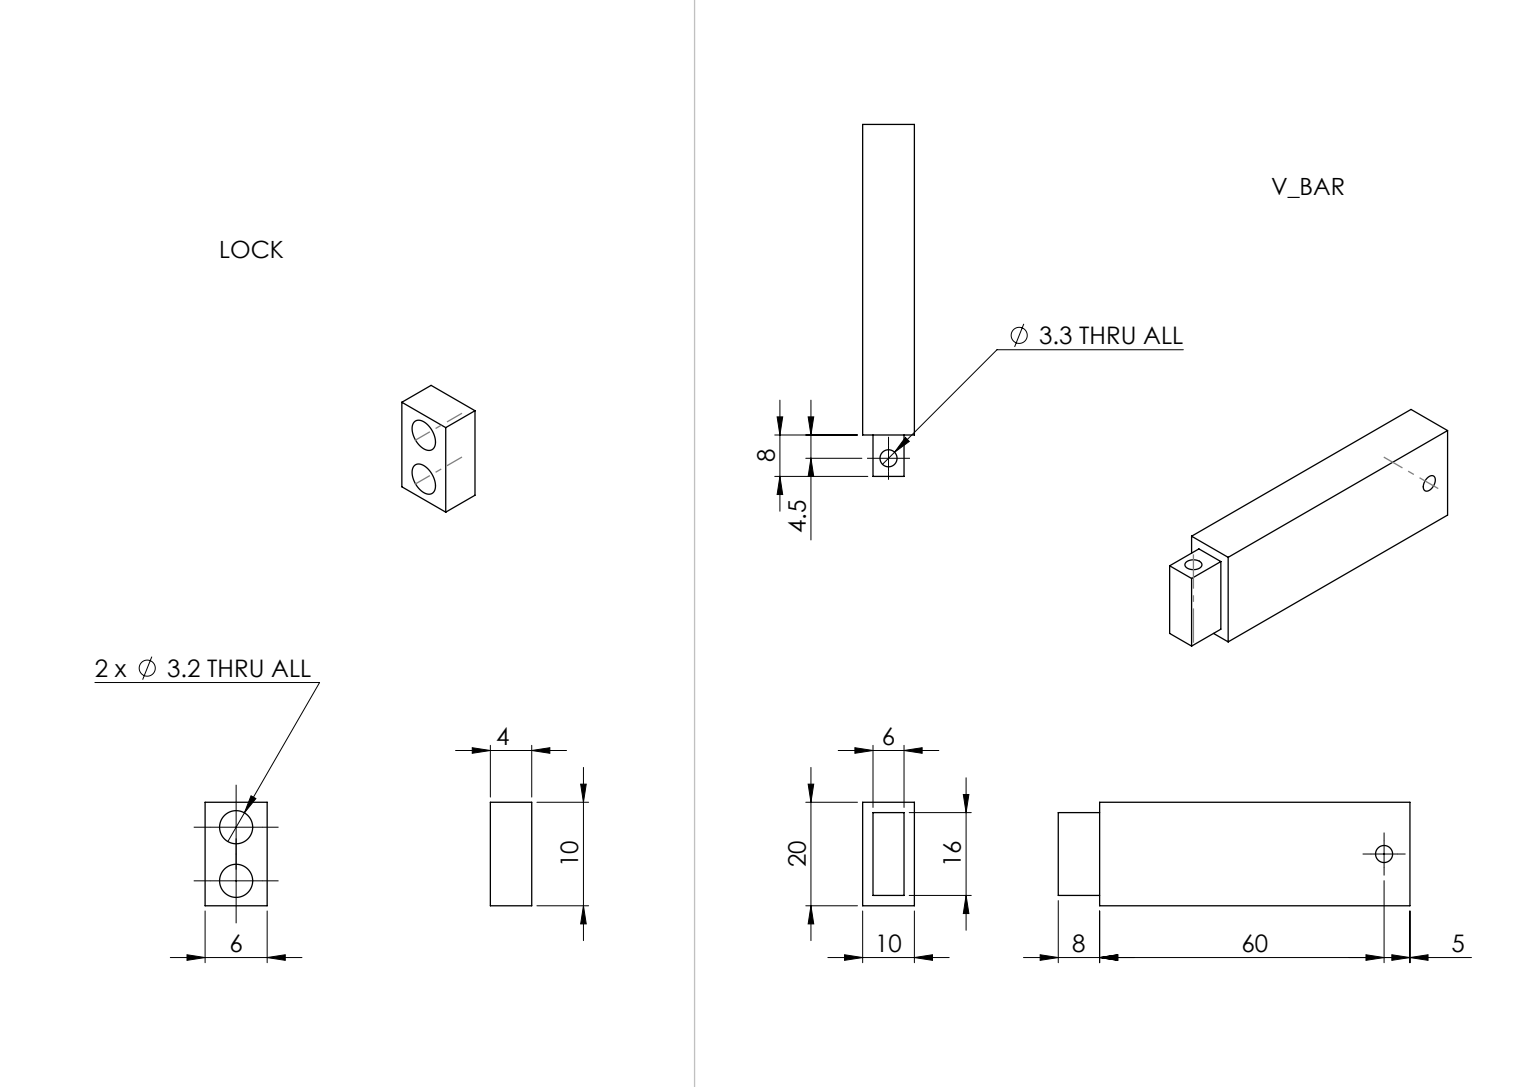
ISO-10303-21;
HEADER;
FILE_DESCRIPTION (('STEP AP214'),
    '1' );
FILE_NAME ('lock.step',
    '2026-10-08T12:12:07',
    ( '' ),
    ( '' ),
    'SwSTEP 2.0',
    'SolidWorks 2026',
    '' );
FILE_SCHEMA (( 'AUTOMOTIVE_DESIGN' ));
ENDSEC;

DATA;
#16=EDGE_LOOP ( 'NONE', ( #282, #7065, #6159, #322 ) ) ;
#17=ADVANCED_FACE ( 'NONE', ( #5328 ), #856, .F. ) ;
#69=CYLINDRICAL_SURFACE ( 'NONE', #6742, 1.599999999999992983 ) ;
#73=EDGE_LOOP ( 'NONE', ( #3445, #4824, #2962, #715 ) ) ;
#74=FACE_OUTER_BOUND ( 'NONE', #4146, .T. ) ;
#91=SURFACE_SIDE_STYLE ('',( #6493 ) ) ;
#113=DIRECTION ( 'NONE',  ( -1.734723475976806848E-16, 1.000000000000000000, -0.000000000000000000 ) ) ;
#141=SURFACE_STYLE_USAGE ( .BOTH. , #5841 ) ;
#160=ORIENTED_EDGE ( 'NONE', *, *, #1858, .F. ) ;
#167=EDGE_CURVE ( 'NONE', #3524, #3495, #1661, .T. ) ;
#171=FACE_BOUND ( 'NONE', #7717, .T. ) ;
#177=CARTESIAN_POINT ( 'NONE',  ( 1.599999999999986988, 42.68016229225776925, 0.000000000000000000 ) ) ;
#236=CARTESIAN_POINT ( 'NONE',  ( -3.000000000000000888, 45.09008114612887397, 4.000000000000000000 ) ) ;
#237=PRODUCT_CONTEXT ( 'NONE', #7877, 'mechanical' ) ;
#282=ORIENTED_EDGE ( 'NONE', *, *, #5845, .T. ) ;
#290=FILL_AREA_STYLE_COLOUR ( '', #5069 ) ;
#322=ORIENTED_EDGE ( 'NONE', *, *, #4660, .T. ) ;
#339=ORIENTED_EDGE ( 'NONE', *, *, #6913, .F. ) ;
#436=( GEOMETRIC_REPRESENTATION_CONTEXT ( 3 ) GLOBAL_UNCERTAINTY_ASSIGNED_CONTEXT ( ( #3628 ) ) GLOBAL_UNIT_ASSIGNED_CONTEXT ( ( #6999, #3191, #7744 ) ) REPRESENTATION_CONTEXT ( 'NONE', 'WORKASPACE' ) );
#515=CARTESIAN_POINT ( 'NONE',  ( -3.000000000000000888, 45.09008114612887397, 4.000000000000000000 ) ) ;
#540=( GEOMETRIC_REPRESENTATION_CONTEXT ( 3 ) GLOBAL_UNCERTAINTY_ASSIGNED_CONTEXT ( ( #3548 ) ) GLOBAL_UNIT_ASSIGNED_CONTEXT ( ( #3306, #2837, #2061 ) ) REPRESENTATION_CONTEXT ( 'NONE', 'WORKASPACE' ) );
#548=LINE ( 'NONE', #1806, #3702 ) ;
#561=DIRECTION ( 'NONE',  ( -0.000000000000000000, -0.000000000000000000, 1.000000000000000000 ) ) ;
#575=LINE ( 'NONE', #3747, #3853 ) ;
#588=EDGE_LOOP ( 'NONE', ( #3671, #2915, #1768, #4961 ) ) ;
#600=PRODUCT ( 'lock', 'lock', '', ( #237 ) ) ;
#604=VERTEX_POINT ( 'NONE', #1255 ) ;
#616=CARTESIAN_POINT ( 'NONE',  ( -1.600000000000010969, 42.68016229225776925, 0.000000000000000000 ) ) ;
#634=ADVANCED_FACE ( 'NONE', ( #74 ), #4574, .F. ) ;
#637=DIRECTION ( 'NONE',  ( -0.000000000000000000, -0.000000000000000000, 1.000000000000000000 ) ) ;
#640=VECTOR ( 'NONE', #5019, 1000.000000000000000 ) ;
#673=ORIENTED_EDGE ( 'NONE', *, *, #2621, .F. ) ;
#715=ORIENTED_EDGE ( 'NONE', *, *, #2234, .T. ) ;
#791=AXIS2_PLACEMENT_3D ( 'NONE', #7600, #2531, #5080 ) ;
#848=DIRECTION ( 'NONE',  ( -0.000000000000000000, -0.000000000000000000, 1.000000000000000000 ) ) ;
#851=CARTESIAN_POINT ( 'NONE',  ( 1.599999999999974998, 42.68016229225776925, 4.000000000000001776 ) ) ;
#856=PLANE ( 'NONE',  #8064 ) ;
#886=ADVANCED_BREP_SHAPE_REPRESENTATION ( '', ( #1401, #1587 ), #3101 ) ;
#911=EDGE_LOOP ( 'NONE', ( #160, #3033, #4699, #339 ) ) ;
#919=FILL_AREA_STYLE ('',( #290 ) ) ;
#1073=EDGE_LOOP ( 'NONE', ( #6447, #5983, #2589, #4040 ) ) ;
#1085=DIRECTION ( 'NONE',  ( 1.000000000000000000, 0.000000000000000000, 0.000000000000000000 ) ) ;
#1124=PRODUCT_DEFINITION_SHAPE ( 'NONE', 'NONE',  #7899 ) ;
#1134=CARTESIAN_POINT ( 'NONE',  ( -1.599999999999986766, 37.49999999999999289, 4.000000000000001776 ) ) ;
#1159=EDGE_CURVE ( 'NONE', #3778, #604, #1443, .T. ) ;
#1179=DIRECTION ( 'NONE',  ( 1.000000000000000000, 0.000000000000000000, 0.000000000000000000 ) ) ;
#1181=CARTESIAN_POINT ( 'NONE',  ( 0.000000000000000000, 37.49999999999999289, 4.000000000000001776 ) ) ;
#1220=DIRECTION ( 'NONE',  ( -0.000000000000000000, -0.000000000000000000, 1.000000000000000000 ) ) ;
#1221=EDGE_LOOP ( 'NONE', ( #5440, #1947 ) ) ;
#1243=DIRECTION ( 'NONE',  ( 1.000000000000000000, 0.000000000000000000, 0.000000000000000000 ) ) ;
#1255=CARTESIAN_POINT ( 'NONE',  ( -3.000000000000000888, 45.09008114612887397, 0.000000000000000000 ) ) ;
#1263=VERTEX_POINT ( 'NONE', #4263 ) ;
#1290=DIRECTION ( 'NONE',  ( -0.000000000000000000, -0.000000000000000000, 1.000000000000000000 ) ) ;
#1294=ORIENTED_EDGE ( 'NONE', *, *, #1938, .F. ) ;
#1300=CARTESIAN_POINT ( 'NONE',  ( 1.599999999999998979, 37.49999999999999289, 0.000000000000000000 ) ) ;
#1326=CIRCLE ( 'NONE', #8075, 1.599999999999998979 ) ;
#1372=AXIS2_PLACEMENT_3D ( 'NONE', #515, #4264, #3549 ) ;
#1378=LINE ( 'NONE', #3393, #1984 ) ;
#1401=MANIFOLD_SOLID_BREP ( 'M3 Clearance Hole1', #6605 ) ;
#1428=ORIENTED_EDGE ( 'NONE', *, *, #3937, .T. ) ;
#1436=AXIS2_PLACEMENT_3D ( 'NONE', #1181, #2518, #6869 ) ;
#1443=LINE ( 'NONE', #5995, #2545 ) ;
#1470=ORIENTED_EDGE ( 'NONE', *, *, #6913, .T. ) ;
#1509=CARTESIAN_POINT ( 'NONE',  ( 0.000000000000000000, 37.49999999999999289, 4.000000000000000000 ) ) ;
#1510=STYLED_ITEM ( 'NONE', ( #7117 ), #886 ) ;
#1568=CIRCLE ( 'NONE', #4360, 1.599999999999998979 ) ;
#1575=VERTEX_POINT ( 'NONE', #6120 ) ;
#1586=AXIS2_PLACEMENT_3D ( 'NONE', #5762, #637, #3188 ) ;
#1587=AXIS2_PLACEMENT_3D ( 'NONE', #3942, #5152, #6454 ) ;
#1594=PLANE ( 'NONE',  #2523 ) ;
#1597=PLANE ( 'NONE',  #7271 ) ;
#1604=MECHANICAL_DESIGN_GEOMETRIC_PRESENTATION_REPRESENTATION('',(#2792),#540);
#1614=DIRECTION ( 'NONE',  ( -1.000000000000000000, -0.000000000000000000, -0.000000000000000000 ) ) ;
#1661=LINE ( 'NONE', #4990, #4757 ) ;
#1693=AXIS2_PLACEMENT_3D ( 'NONE', #1509, #7116, #2715 ) ;
#1706=LINE ( 'NONE', #4240, #4219 ) ;
#1736=PLANE ( 'NONE',  #1372 ) ;
#1768=ORIENTED_EDGE ( 'NONE', *, *, #5700, .F. ) ;
#1777=CARTESIAN_POINT ( 'NONE',  ( 1.599999999999992983, 37.49999999999999289, 4.000000000000000000 ) ) ;
#1804=CARTESIAN_POINT ( 'NONE',  ( -1.198153218366585720E-14, 42.68016229225776925, 4.000000000000001776 ) ) ;
#1806=CARTESIAN_POINT ( 'NONE',  ( -2.999999999999998668, 35.09008114612887397, 4.000000000000000000 ) ) ;
#1829=DIRECTION ( 'NONE',  ( 1.000000000000000000, 0.000000000000000000, 0.000000000000000000 ) ) ;
#1847=DIRECTION ( 'NONE',  ( -0.000000000000000000, -0.000000000000000000, -1.000000000000000000 ) ) ;
#1858=EDGE_CURVE ( 'NONE', #2626, #5387, #2479, .T. ) ;
#1938=EDGE_CURVE ( 'NONE', #5254, #604, #6760, .T. ) ;
#1941=EDGE_LOOP ( 'NONE', ( #6862, #6850 ) ) ;
#1943=CYLINDRICAL_SURFACE ( 'NONE', #1586, 1.599999999999992983 ) ;
#1947=ORIENTED_EDGE ( 'NONE', *, *, #3242, .F. ) ;
#1972=DIRECTION ( 'NONE',  ( 1.000000000000000000, 0.000000000000000000, 0.000000000000000000 ) ) ;
#1975=VERTEX_POINT ( 'NONE', #3071 ) ;
#1984=VECTOR ( 'NONE', #113, 1000.000000000000000 ) ;
#2021=ORIENTED_EDGE ( 'NONE', *, *, #5845, .F. ) ;
#2061=( NAMED_UNIT ( * ) SI_UNIT ( $, .STERADIAN. ) SOLID_ANGLE_UNIT ( ) );
#2093=FACE_OUTER_BOUND ( 'NONE', #5244, .T. ) ;
#2185=CYLINDRICAL_SURFACE ( 'NONE', #6874, 1.599999999999992983 ) ;
#2212=DIRECTION ( 'NONE',  ( 1.734723475976806848E-16, -1.000000000000000000, 0.000000000000000000 ) ) ;
#2224=CARTESIAN_POINT ( 'NONE',  ( -1.198153218366585720E-14, 42.68016229225776925, 4.000000000000000000 ) ) ;
#2234=EDGE_CURVE ( 'NONE', #2468, #1975, #4424, .T. ) ;
#2259=ADVANCED_FACE ( 'NONE', ( #6256 ), #1736, .F. ) ;
#2272=FACE_OUTER_BOUND ( 'NONE', #2603, .T. ) ;
#2297=FACE_BOUND ( 'NONE', #6331, .T. ) ;
#2468=VERTEX_POINT ( 'NONE', #851 ) ;
#2479=CIRCLE ( 'NONE', #3151, 1.599999999999998979 ) ;
#2486=ORIENTED_EDGE ( 'NONE', *, *, #4341, .T. ) ;
#2518=DIRECTION ( 'NONE',  ( -0.000000000000000000, -0.000000000000000000, 1.000000000000000000 ) ) ;
#2523=AXIS2_PLACEMENT_3D ( 'NONE', #3499, #5906, #7771 ) ;
#2531=DIRECTION ( 'NONE',  ( -0.000000000000000000, -0.000000000000000000, 1.000000000000000000 ) ) ;
#2545=VECTOR ( 'NONE', #4053, 1000.000000000000000 ) ;
#2589=ORIENTED_EDGE ( 'NONE', *, *, #5700, .T. ) ;
#2603=EDGE_LOOP ( 'NONE', ( #5942, #1428, #4473, #6361 ) ) ;
#2621=EDGE_CURVE ( 'NONE', #2626, #4815, #5978, .T. ) ;
#2626=VERTEX_POINT ( 'NONE', #7513 ) ;
#2666=AXIS2_PLACEMENT_3D ( 'NONE', #1804, #3289, #3221 ) ;
#2697=PRODUCT_DEFINITION_FORMATION_WITH_SPECIFIED_SOURCE ( 'ANY', '', #600, .NOT_KNOWN. ) ;
#2715=DIRECTION ( 'NONE',  ( 1.000000000000000000, 0.000000000000000000, 0.000000000000000000 ) ) ;
#2792=STYLED_ITEM ( 'NONE', ( #2800 ), #1401 ) ;
#2800=PRESENTATION_STYLE_ASSIGNMENT (( #141 ) ) ;
#2820=VERTEX_POINT ( 'NONE', #3831 ) ;
#2822=DIRECTION ( 'NONE',  ( 1.000000000000000000, 2.168404344971008621E-16, -0.000000000000000000 ) ) ;
#2827=DIRECTION ( 'NONE',  ( -0.000000000000000000, -0.000000000000000000, 1.000000000000000000 ) ) ;
#2837=( NAMED_UNIT ( * ) PLANE_ANGLE_UNIT ( ) SI_UNIT ( $, .RADIAN. ) );
#2852=CARTESIAN_POINT ( 'NONE',  ( -1.198153218366585720E-14, 42.68016229225776925, 0.000000000000000000 ) ) ;
#2915=ORIENTED_EDGE ( 'NONE', *, *, #3565, .F. ) ;
#2959=UNCERTAINTY_MEASURE_WITH_UNIT (LENGTH_MEASURE( 1.000000000000000082E-05 ), #5067, 'distance_accuracy_value', 'NONE');
#2962=ORIENTED_EDGE ( 'NONE', *, *, #2989, .T. ) ;
#2989=EDGE_CURVE ( 'NONE', #8142, #2468, #6668, .T. ) ;
#3033=ORIENTED_EDGE ( 'NONE', *, *, #2621, .T. ) ;
#3042=VECTOR ( 'NONE', #1614, 1000.000000000000000 ) ;
#3071=CARTESIAN_POINT ( 'NONE',  ( -1.599999999999998757, 42.68016229225776925, 4.000000000000001776 ) ) ;
#3078=CARTESIAN_POINT ( 'NONE',  ( 0.000000000000000000, 37.49999999999999289, 0.000000000000000000 ) ) ;
#3091=ORIENTED_EDGE ( 'NONE', *, *, #1938, .T. ) ;
#3101=( GEOMETRIC_REPRESENTATION_CONTEXT ( 3 ) GLOBAL_UNCERTAINTY_ASSIGNED_CONTEXT ( ( #2959 ) ) GLOBAL_UNIT_ASSIGNED_CONTEXT ( ( #5067, #4299, #4469 ) ) REPRESENTATION_CONTEXT ( 'NONE', 'WORKASPACE' ) );
#3139=FACE_OUTER_BOUND ( 'NONE', #911, .T. ) ;
#3151=AXIS2_PLACEMENT_3D ( 'NONE', #5650, #3651, #1243 ) ;
#3152=LINE ( 'NONE', #1777, #640 ) ;
#3186=VECTOR ( 'NONE', #3506, 1000.000000000000000 ) ;
#3188=DIRECTION ( 'NONE',  ( 1.000000000000000000, 0.000000000000000000, 0.000000000000000000 ) ) ;
#3191=( NAMED_UNIT ( * ) PLANE_ANGLE_UNIT ( ) SI_UNIT ( $, .RADIAN. ) );
#3221=DIRECTION ( 'NONE',  ( 1.000000000000000000, 0.000000000000000000, 0.000000000000000000 ) ) ;
#3242=EDGE_CURVE ( 'NONE', #4815, #1263, #3832, .T. ) ;
#3284=ORIENTED_EDGE ( 'NONE', *, *, #4538, .F. ) ;
#3289=DIRECTION ( 'NONE',  ( -0.000000000000000000, -0.000000000000000000, 1.000000000000000000 ) ) ;
#3306=( LENGTH_UNIT ( ) NAMED_UNIT ( * ) SI_UNIT ( .MILLI., .METRE. ) );
#3313=ADVANCED_FACE ( 'NONE', ( #2093 ), #4554, .F. ) ;
#3393=CARTESIAN_POINT ( 'NONE',  ( 2.999999999999999112, 45.09008114612887397, 0.000000000000000000 ) ) ;
#3445=ORIENTED_EDGE ( 'NONE', *, *, #3937, .F. ) ;
#3495=VERTEX_POINT ( 'NONE', #7397 ) ;
#3496=ADVANCED_FACE ( 'NONE', ( #4126, #2297, #7273 ), #1597, .T. ) ;
#3499=CARTESIAN_POINT ( 'NONE',  ( 0.000000000000000000, 0.000000000000000000, 0.000000000000000000 ) ) ;
#3506=DIRECTION ( 'NONE',  ( -0.000000000000000000, -0.000000000000000000, -1.000000000000000000 ) ) ;
#3524=VERTEX_POINT ( 'NONE', #5500 ) ;
#3548=UNCERTAINTY_MEASURE_WITH_UNIT (LENGTH_MEASURE( 1.000000000000000082E-05 ), #3306, 'distance_accuracy_value', 'NONE');
#3549=DIRECTION ( 'NONE',  ( 0.000000000000000000, -0.000000000000000000, -1.000000000000000000 ) ) ;
#3565=EDGE_CURVE ( 'NONE', #3851, #3524, #548, .T. ) ;
#3586=CARTESIAN_POINT ( 'NONE',  ( 2.999999999999999112, 45.09008114612887397, 0.000000000000000000 ) ) ;
#3613=EDGE_CURVE ( 'NONE', #3962, #8142, #7676, .T. ) ;
#3628=UNCERTAINTY_MEASURE_WITH_UNIT (LENGTH_MEASURE( 1.000000000000000082E-05 ), #6999, 'distance_accuracy_value', 'NONE');
#3651=DIRECTION ( 'NONE',  ( -0.000000000000000000, -0.000000000000000000, 1.000000000000000000 ) ) ;
#3671=ORIENTED_EDGE ( 'NONE', *, *, #4538, .T. ) ;
#3699=CARTESIAN_POINT ( 'NONE',  ( -1.198153218366585720E-14, 42.68016229225776925, 4.000000000000000000 ) ) ;
#3702=VECTOR ( 'NONE', #1847, 1000.000000000000000 ) ;
#3704=AXIS2_PLACEMENT_3D ( 'NONE', #5303, #7164, #2212 ) ;
#3747=CARTESIAN_POINT ( 'NONE',  ( -3.000000000000000888, 45.09008114612887397, 0.000000000000000000 ) ) ;
#3756=PRODUCT_DEFINITION_CONTEXT ( 'detailed design', #5776, 'design' ) ;
#3778=VERTEX_POINT ( 'NONE', #236 ) ;
#3788=ORIENTED_EDGE ( 'NONE', *, *, #3613, .T. ) ;
#3792=CARTESIAN_POINT ( 'NONE',  ( -3.000000000000000888, 45.09008114612887397, 4.000000000000000000 ) ) ;
#3831=CARTESIAN_POINT ( 'NONE',  ( 2.999999999999999112, 45.09008114612887397, 4.000000000000000000 ) ) ;
#3832=CIRCLE ( 'NONE', #1436, 1.599999999999986766 ) ;
#3851=VERTEX_POINT ( 'NONE', #4697 ) ;
#3853=VECTOR ( 'NONE', #7746, 1000.000000000000000 ) ;
#3896=AXIS2_PLACEMENT_3D ( 'NONE', #7541, #561, #5641 ) ;
#3937=EDGE_CURVE ( 'NONE', #3962, #1975, #1706, .T. ) ;
#3942=CARTESIAN_POINT ( 'NONE',  ( 0.000000000000000000, 0.000000000000000000, 0.000000000000000000 ) ) ;
#3956=ORIENTED_EDGE ( 'NONE', *, *, #7943, .T. ) ;
#3962=VERTEX_POINT ( 'NONE', #616 ) ;
#3971=FILL_AREA_STYLE_COLOUR ( '', #7994 ) ;
#4040=ORIENTED_EDGE ( 'NONE', *, *, #4829, .T. ) ;
#4053=DIRECTION ( 'NONE',  ( -0.000000000000000000, -0.000000000000000000, -1.000000000000000000 ) ) ;
#4106=ORIENTED_EDGE ( 'NONE', *, *, #4660, .F. ) ;
#4126=FACE_BOUND ( 'NONE', #1221, .T. ) ;
#4146=EDGE_LOOP ( 'NONE', ( #7368, #4106, #5410, #7728 ) ) ;
#4219=VECTOR ( 'NONE', #2827, 1000.000000000000000 ) ;
#4222=DIRECTION ( 'NONE',  ( -0.000000000000000000, -0.000000000000000000, 1.000000000000000000 ) ) ;
#4240=CARTESIAN_POINT ( 'NONE',  ( -1.600000000000004752, 42.68016229225776925, 4.000000000000000000 ) ) ;
#4263=CARTESIAN_POINT ( 'NONE',  ( 1.599999999999986766, 37.49999999999999289, 4.000000000000001776 ) ) ;
#4264=DIRECTION ( 'NONE',  ( 0.000000000000000000, -1.000000000000000000, 0.000000000000000000 ) ) ;
#4273=CARTESIAN_POINT ( 'NONE',  ( -3.000000000000000888, 45.09008114612887397, 0.000000000000000000 ) ) ;
#4298=CARTESIAN_POINT ( 'NONE',  ( 2.999999999999999112, 45.09008114612887397, 4.000000000000000000 ) ) ;
#4299=( NAMED_UNIT ( * ) PLANE_ANGLE_UNIT ( ) SI_UNIT ( $, .RADIAN. ) );
#4334=ORIENTED_EDGE ( 'NONE', *, *, #7613, .F. ) ;
#4341=EDGE_CURVE ( 'NONE', #1263, #4815, #6900, .T. ) ;
#4360=AXIS2_PLACEMENT_3D ( 'NONE', #3078, #4409, #4488 ) ;
#4362=LINE ( 'NONE', #3792, #7924 ) ;
#4405=ORIENTED_EDGE ( 'NONE', *, *, #1159, .F. ) ;
#4409=DIRECTION ( 'NONE',  ( -0.000000000000000000, -0.000000000000000000, 1.000000000000000000 ) ) ;
#4424=CIRCLE ( 'NONE', #3896, 1.599999999999986766 ) ;
#4435=MECHANICAL_DESIGN_GEOMETRIC_PRESENTATION_REPRESENTATION('',(#1510),#436);
#4455=DIRECTION ( 'NONE',  ( 0.000000000000000000, 1.000000000000000000, 0.000000000000000000 ) ) ;
#4469=( NAMED_UNIT ( * ) SI_UNIT ( $, .STERADIAN. ) SOLID_ANGLE_UNIT ( ) );
#4473=ORIENTED_EDGE ( 'NONE', *, *, #7613, .T. ) ;
#4488=DIRECTION ( 'NONE',  ( 1.000000000000000000, 0.000000000000000000, 0.000000000000000000 ) ) ;
#4500=CARTESIAN_POINT ( 'NONE',  ( -1.198153218366585720E-14, 42.68016229225776925, 0.000000000000000000 ) ) ;
#4538=EDGE_CURVE ( 'NONE', #604, #3524, #575, .T. ) ;
#4554=CYLINDRICAL_SURFACE ( 'NONE', #1693, 1.599999999999992983 ) ;
#4556=SHAPE_REPRESENTATION_RELATIONSHIP ( 'NONE' , 'NONE' ,  #7239, #886 ) ;
#4574=PLANE ( 'NONE',  #5189 ) ;
#4619=EDGE_LOOP ( 'NONE', ( #2021, #4723, #3284, #1294 ) ) ;
#4633=PLANE ( 'NONE',  #3704 ) ;
#4660=EDGE_CURVE ( 'NONE', #1575, #3495, #5912, .T. ) ;
#4661=ADVANCED_FACE ( 'NONE', ( #6497 ), #4633, .F. ) ;
#4671=VECTOR ( 'NONE', #6639, 1000.000000000000000 ) ;
#4697=CARTESIAN_POINT ( 'NONE',  ( -2.999999999999998668, 35.09008114612887397, 4.000000000000000000 ) ) ;
#4699=ORIENTED_EDGE ( 'NONE', *, *, #3242, .T. ) ;
#4723=ORIENTED_EDGE ( 'NONE', *, *, #167, .F. ) ;
#4729=LINE ( 'NONE', #4817, #7014 ) ;
#4757=VECTOR ( 'NONE', #1829, 1000.000000000000000 ) ;
#4776=CARTESIAN_POINT ( 'NONE',  ( -3.000000000000000888, 45.09008114612887397, 4.000000000000000000 ) ) ;
#4815=VERTEX_POINT ( 'NONE', #1134 ) ;
#4817=CARTESIAN_POINT ( 'NONE',  ( 2.999999999999999112, 45.09008114612887397, 4.000000000000000000 ) ) ;
#4824=ORIENTED_EDGE ( 'NONE', *, *, #7943, .F. ) ;
#4829=EDGE_CURVE ( 'NONE', #3851, #1575, #7361, .T. ) ;
#4832=CARTESIAN_POINT ( 'NONE',  ( 0.000000000000000000, 0.000000000000000000, 4.000000000000000000 ) ) ;
#4961=ORIENTED_EDGE ( 'NONE', *, *, #1159, .T. ) ;
#4990=CARTESIAN_POINT ( 'NONE',  ( -2.999999999999998668, 35.09008114612887397, 0.000000000000000000 ) ) ;
#5019=DIRECTION ( 'NONE',  ( -0.000000000000000000, -0.000000000000000000, 1.000000000000000000 ) ) ;
#5022=ADVANCED_FACE ( 'NONE', ( #3139 ), #1943, .F. ) ;
#5030=DIRECTION ( 'NONE',  ( -1.000000000000000000, -0.000000000000000000, -0.000000000000000000 ) ) ;
#5067=( LENGTH_UNIT ( ) NAMED_UNIT ( * ) SI_UNIT ( .MILLI., .METRE. ) );
#5069=COLOUR_RGB ( '', 0.31764706, 0.68627451, 0.89019608) ;
#5080=DIRECTION ( 'NONE',  ( 1.000000000000000000, 0.000000000000000000, 0.000000000000000000 ) ) ;
#5092=CARTESIAN_POINT ( 'NONE',  ( -2.999999999999998668, 35.09008114612887397, 4.000000000000000000 ) ) ;
#5104=ADVANCED_FACE ( 'NONE', ( #7888, #171, #6489 ), #1594, .F. ) ;
#5110=FILL_AREA_STYLE ('',( #3971 ) ) ;
#5152=DIRECTION ( 'NONE',  ( 0.000000000000000000, 0.000000000000000000, 1.000000000000000000 ) ) ;
#5189=AXIS2_PLACEMENT_3D ( 'NONE', #5092, #4455, #5663 ) ;
#5244=EDGE_LOOP ( 'NONE', ( #673, #7650, #1470, #2486 ) ) ;
#5254=VERTEX_POINT ( 'NONE', #3586 ) ;
#5303=CARTESIAN_POINT ( 'NONE',  ( 2.999999999999999112, 45.09008114612887397, 4.000000000000000000 ) ) ;
#5328=FACE_OUTER_BOUND ( 'NONE', #588, .T. ) ;
#5369=SHAPE_DEFINITION_REPRESENTATION ( #1124, #7239 ) ;
#5387=VERTEX_POINT ( 'NONE', #1300 ) ;
#5393=DIRECTION ( 'NONE',  ( 1.000000000000000000, 0.000000000000000000, 0.000000000000000000 ) ) ;
#5410=ORIENTED_EDGE ( 'NONE', *, *, #4829, .F. ) ;
#5423=AXIS2_PLACEMENT_3D ( 'NONE', #4500, #1220, #1972 ) ;
#5440=ORIENTED_EDGE ( 'NONE', *, *, #4341, .F. ) ;
#5500=CARTESIAN_POINT ( 'NONE',  ( -2.999999999999998668, 35.09008114612887397, 0.000000000000000000 ) ) ;
#5641=DIRECTION ( 'NONE',  ( 1.000000000000000000, 0.000000000000000000, 0.000000000000000000 ) ) ;
#5650=CARTESIAN_POINT ( 'NONE',  ( 0.000000000000000000, 37.49999999999999289, 0.000000000000000000 ) ) ;
#5663=DIRECTION ( 'NONE',  ( 0.000000000000000000, -0.000000000000000000, 1.000000000000000000 ) ) ;
#5674=EDGE_LOOP ( 'NONE', ( #3091, #4405, #6155, #6801 ) ) ;
#5700=EDGE_CURVE ( 'NONE', #3778, #3851, #4362, .T. ) ;
#5713=VECTOR ( 'NONE', #1179, 1000.000000000000000 ) ;
#5762=CARTESIAN_POINT ( 'NONE',  ( 0.000000000000000000, 37.49999999999999289, 4.000000000000000000 ) ) ;
#5776=APPLICATION_CONTEXT ( 'automotive_design' ) ;
#5783=ADVANCED_FACE ( 'NONE', ( #7016 ), #69, .F. ) ;
#5815=EDGE_CURVE ( 'NONE', #5387, #2626, #1568, .T. ) ;
#5841=SURFACE_SIDE_STYLE ('',( #7158 ) ) ;
#5845=EDGE_CURVE ( 'NONE', #3495, #5254, #1378, .T. ) ;
#5906=DIRECTION ( 'NONE',  ( -0.000000000000000000, 0.000000000000000000, 1.000000000000000000 ) ) ;
#5912=LINE ( 'NONE', #6612, #3186 ) ;
#5942=ORIENTED_EDGE ( 'NONE', *, *, #3613, .F. ) ;
#5978=LINE ( 'NONE', #7881, #4671 ) ;
#5983=ORIENTED_EDGE ( 'NONE', *, *, #7948, .T. ) ;
#5995=CARTESIAN_POINT ( 'NONE',  ( -3.000000000000000888, 45.09008114612887397, 4.000000000000000000 ) ) ;
#6034=ADVANCED_FACE ( 'NONE', ( #2272 ), #2185, .F. ) ;
#6043=DIRECTION ( 'NONE',  ( -0.000000000000000000, -0.000000000000000000, 1.000000000000000000 ) ) ;
#6120=CARTESIAN_POINT ( 'NONE',  ( 3.000000000000000888, 35.09008114612887397, 4.000000000000000000 ) ) ;
#6124=DIRECTION ( 'NONE',  ( -0.000000000000000000, -0.000000000000000000, -1.000000000000000000 ) ) ;
#6155=ORIENTED_EDGE ( 'NONE', *, *, #7948, .F. ) ;
#6159=ORIENTED_EDGE ( 'NONE', *, *, #6362, .F. ) ;
#6160=CARTESIAN_POINT ( 'NONE',  ( -2.999999999999998668, 35.09008114612887397, 4.000000000000000000 ) ) ;
#6200=LINE ( 'NONE', #4298, #7423 ) ;
#6256=FACE_OUTER_BOUND ( 'NONE', #5674, .T. ) ;
#6274=DIRECTION ( 'NONE',  ( 1.000000000000000000, 0.000000000000000000, 0.000000000000000000 ) ) ;
#6331=EDGE_LOOP ( 'NONE', ( #6404, #4334 ) ) ;
#6361=ORIENTED_EDGE ( 'NONE', *, *, #2989, .F. ) ;
#6362=EDGE_CURVE ( 'NONE', #1575, #2820, #4729, .T. ) ;
#6380=CIRCLE ( 'NONE', #2666, 1.599999999999986766 ) ;
#6404=ORIENTED_EDGE ( 'NONE', *, *, #2234, .F. ) ;
#6447=ORIENTED_EDGE ( 'NONE', *, *, #6362, .T. ) ;
#6454=DIRECTION ( 'NONE',  ( 1.000000000000000000, 0.000000000000000000, 0.000000000000000000 ) ) ;
#6489=FACE_OUTER_BOUND ( 'NONE', #4619, .T. ) ;
#6493=SURFACE_STYLE_FILL_AREA ( #5110 ) ;
#6497=FACE_OUTER_BOUND ( 'NONE', #16, .T. ) ;
#6542=CARTESIAN_POINT ( 'NONE',  ( 1.599999999999980993, 42.68016229225776925, 4.000000000000000000 ) ) ;
#6605=CLOSED_SHELL ( 'NONE', ( #5022, #6034, #4661, #2259, #17, #634, #3496, #5104, #5783, #3313 ) ) ;
#6612=CARTESIAN_POINT ( 'NONE',  ( 3.000000000000000888, 35.09008114612887397, 4.000000000000000000 ) ) ;
#6639=DIRECTION ( 'NONE',  ( -0.000000000000000000, -0.000000000000000000, 1.000000000000000000 ) ) ;
#6651=DIRECTION ( 'NONE',  ( -0.000000000000000000, 0.000000000000000000, 1.000000000000000000 ) ) ;
#6668=LINE ( 'NONE', #6542, #7398 ) ;
#6670=CARTESIAN_POINT ( 'NONE',  ( -3.000000000000000888, 45.09008114612887397, 4.000000000000000000 ) ) ;
#6742=AXIS2_PLACEMENT_3D ( 'NONE', #3699, #1290, #6274 ) ;
#6760=LINE ( 'NONE', #4273, #7379 ) ;
#6801=ORIENTED_EDGE ( 'NONE', *, *, #7233, .T. ) ;
#6850=ORIENTED_EDGE ( 'NONE', *, *, #1858, .T. ) ;
#6862=ORIENTED_EDGE ( 'NONE', *, *, #5815, .T. ) ;
#6869=DIRECTION ( 'NONE',  ( 1.000000000000000000, 0.000000000000000000, 0.000000000000000000 ) ) ;
#6874=AXIS2_PLACEMENT_3D ( 'NONE', #2224, #6043, #8031 ) ;
#6900=CIRCLE ( 'NONE', #791, 1.599999999999986766 ) ;
#6913=EDGE_CURVE ( 'NONE', #5387, #1263, #3152, .T. ) ;
#6999=( LENGTH_UNIT ( ) NAMED_UNIT ( * ) SI_UNIT ( .MILLI., .METRE. ) );
#7014=VECTOR ( 'NONE', #7347, 1000.000000000000000 ) ;
#7016=FACE_OUTER_BOUND ( 'NONE', #73, .T. ) ;
#7065=ORIENTED_EDGE ( 'NONE', *, *, #7233, .F. ) ;
#7116=DIRECTION ( 'NONE',  ( -0.000000000000000000, -0.000000000000000000, 1.000000000000000000 ) ) ;
#7117=PRESENTATION_STYLE_ASSIGNMENT (( #7627 ) ) ;
#7158=SURFACE_STYLE_FILL_AREA ( #919 ) ;
#7164=DIRECTION ( 'NONE',  ( -1.000000000000000000, -1.734723475976806848E-16, 0.000000000000000000 ) ) ;
#7233=EDGE_CURVE ( 'NONE', #2820, #5254, #6200, .T. ) ;
#7239=SHAPE_REPRESENTATION ( 'lock', ( #1587 ), #3101 ) ;
#7271=AXIS2_PLACEMENT_3D ( 'NONE', #4832, #6651, #1085 ) ;
#7273=FACE_OUTER_BOUND ( 'NONE', #1073, .T. ) ;
#7298=LINE ( 'NONE', #6670, #3042 ) ;
#7307=DIRECTION ( 'NONE',  ( -2.168404344971008621E-16, 1.000000000000000000, 0.000000000000000000 ) ) ;
#7347=DIRECTION ( 'NONE',  ( -1.734723475976806848E-16, 1.000000000000000000, -0.000000000000000000 ) ) ;
#7361=LINE ( 'NONE', #6160, #5713 ) ;
#7368=ORIENTED_EDGE ( 'NONE', *, *, #167, .T. ) ;
#7379=VECTOR ( 'NONE', #5030, 1000.000000000000000 ) ;
#7397=CARTESIAN_POINT ( 'NONE',  ( 3.000000000000000888, 35.09008114612887397, 0.000000000000000000 ) ) ;
#7398=VECTOR ( 'NONE', #848, 1000.000000000000000 ) ;
#7423=VECTOR ( 'NONE', #6124, 1000.000000000000000 ) ;
#7513=CARTESIAN_POINT ( 'NONE',  ( -1.599999999999998979, 37.49999999999999289, 0.000000000000000000 ) ) ;
#7541=CARTESIAN_POINT ( 'NONE',  ( -1.198153218366585720E-14, 42.68016229225776925, 4.000000000000001776 ) ) ;
#7600=CARTESIAN_POINT ( 'NONE',  ( 0.000000000000000000, 37.49999999999999289, 4.000000000000001776 ) ) ;
#7613=EDGE_CURVE ( 'NONE', #1975, #2468, #6380, .T. ) ;
#7627=SURFACE_STYLE_USAGE ( .BOTH. , #91 ) ;
#7650=ORIENTED_EDGE ( 'NONE', *, *, #5815, .F. ) ;
#7676=CIRCLE ( 'NONE', #5423, 1.599999999999998979 ) ;
#7717=EDGE_LOOP ( 'NONE', ( #3956, #3788 ) ) ;
#7728=ORIENTED_EDGE ( 'NONE', *, *, #3565, .T. ) ;
#7744=( NAMED_UNIT ( * ) SI_UNIT ( $, .STERADIAN. ) SOLID_ANGLE_UNIT ( ) );
#7746=DIRECTION ( 'NONE',  ( 2.168404344971008621E-16, -1.000000000000000000, 0.000000000000000000 ) ) ;
#7771=DIRECTION ( 'NONE',  ( 1.000000000000000000, 0.000000000000000000, 0.000000000000000000 ) ) ;
#7877=APPLICATION_CONTEXT ( 'automotive_design' ) ;
#7881=CARTESIAN_POINT ( 'NONE',  ( -1.599999999999992983, 37.49999999999999289, 4.000000000000000000 ) ) ;
#7888=FACE_BOUND ( 'NONE', #1941, .T. ) ;
#7899=PRODUCT_DEFINITION ( 'UNKNOWN', '', #2697, #3756 ) ;
#7924=VECTOR ( 'NONE', #8171, 1000.000000000000000 ) ;
#7943=EDGE_CURVE ( 'NONE', #8142, #3962, #1326, .T. ) ;
#7948=EDGE_CURVE ( 'NONE', #2820, #3778, #7298, .T. ) ;
#7994=COLOUR_RGB ( '', 0.31764706, 0.68627451, 0.89019608) ;
#8031=DIRECTION ( 'NONE',  ( 1.000000000000000000, 0.000000000000000000, 0.000000000000000000 ) ) ;
#8064=AXIS2_PLACEMENT_3D ( 'NONE', #4776, #2822, #7307 ) ;
#8075=AXIS2_PLACEMENT_3D ( 'NONE', #2852, #4222, #5393 ) ;
#8142=VERTEX_POINT ( 'NONE', #177 ) ;
#8171=DIRECTION ( 'NONE',  ( 2.168404344971008621E-16, -1.000000000000000000, 0.000000000000000000 ) ) ;
ENDSEC;
END-ISO-10303-21;
